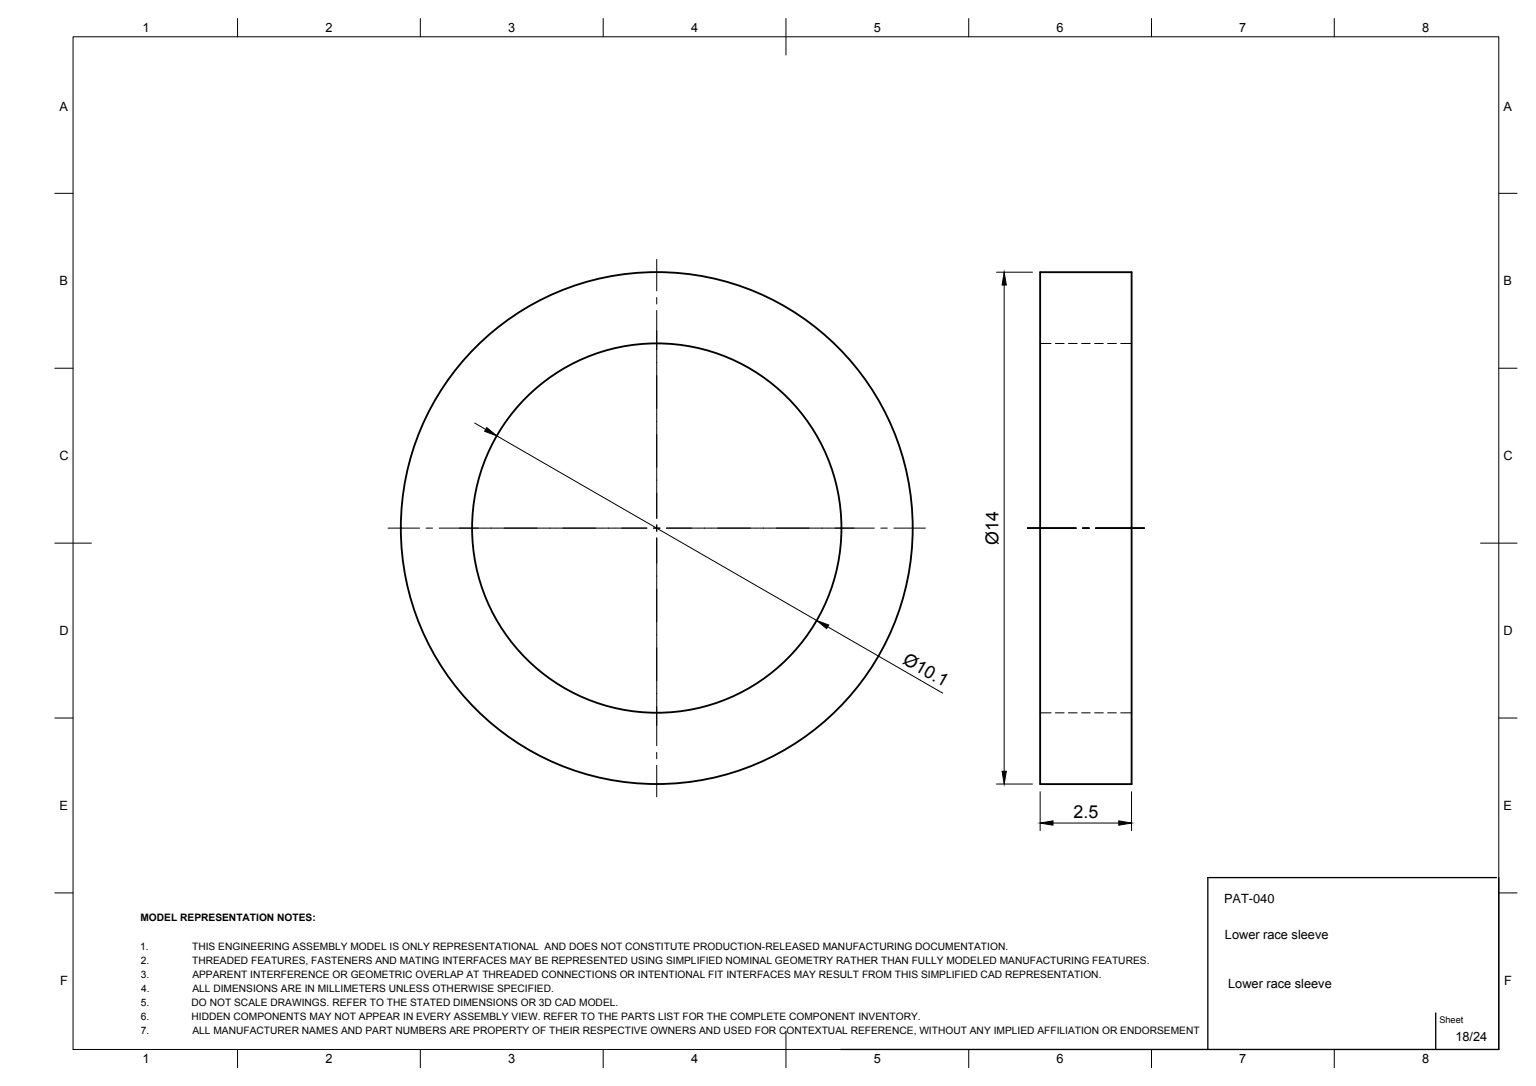
ISO-10303-21;
HEADER;
/* Generated by software containing ST-Developer
 * from STEP Tools, Inc. (www.steptools.com) 
 */

FILE_DESCRIPTION(
/* description */ ('Four-bar tabletop demonstrator'),
/* implementation_level */ '2;1');

FILE_NAME(
/* name */ 'Lower race sleeve.step',
/* time_stamp */ '2026-10-29T17:05:23-07:00',
/* author */ (''),
/* organization */ (''),
/* preprocessor_version */ 'ST-DEVELOPER v20.2',
/* originating_system */ 'Autodesk Translation Framework v15.17.0.0',
/* authorisation */ '');

FILE_SCHEMA (('AUTOMOTIVE_DESIGN { 1 0 10303 214 3 1 1 }'));
ENDSEC;

DATA;
#10=MECHANICAL_DESIGN_GEOMETRIC_PRESENTATION_REPRESENTATION('',(#357),#6705);
#319=SHAPE_REPRESENTATION_RELATIONSHIP('SRR','None',#6829,#334);
#334=ADVANCED_BREP_SHAPE_REPRESENTATION('',(#378),#6702);
#357=STYLED_ITEM('',(#6975),#378);
#378=MANIFOLD_SOLID_BREP('Body1',#3403);
#455=FACE_BOUND('',#1023,.T.);
#456=FACE_BOUND('',#1025,.T.);
#547=PLANE('',#4004);
#548=PLANE('',#4005);
#743=FACE_OUTER_BOUND('',#1020,.T.);
#744=FACE_OUTER_BOUND('',#1021,.T.);
#745=FACE_OUTER_BOUND('',#1022,.T.);
#746=FACE_OUTER_BOUND('',#1024,.T.);
#1020=EDGE_LOOP('',(#3014,#3015,#3016,#3017));
#1021=EDGE_LOOP('',(#3018,#3019,#3020,#3021));
#1022=EDGE_LOOP('',(#3022));
#1023=EDGE_LOOP('',(#3023));
#1024=EDGE_LOOP('',(#3024));
#1025=EDGE_LOOP('',(#3025));
#1192=LINE('',#6475,#1362);
#1193=LINE('',#6481,#1363);
#1362=VECTOR('',#5065,0.505);
#1363=VECTOR('',#5072,0.7);
#1587=CIRCLE('',#3999,0.505);
#1588=CIRCLE('',#4000,0.505);
#1589=CIRCLE('',#4002,0.7);
#1590=CIRCLE('',#4003,0.7);
#1850=VERTEX_POINT('',#6472);
#1851=VERTEX_POINT('',#6474);
#1852=VERTEX_POINT('',#6478);
#1853=VERTEX_POINT('',#6480);
#2243=EDGE_CURVE('',#1850,#1850,#1587,.T.);
#2244=EDGE_CURVE('',#1850,#1851,#1192,.T.);
#2245=EDGE_CURVE('',#1851,#1851,#1588,.T.);
#2246=EDGE_CURVE('',#1852,#1852,#1589,.T.);
#2247=EDGE_CURVE('',#1852,#1853,#1193,.T.);
#2248=EDGE_CURVE('',#1853,#1853,#1590,.T.);
#3014=ORIENTED_EDGE('',*,*,#2243,.F.);
#3015=ORIENTED_EDGE('',*,*,#2244,.T.);
#3016=ORIENTED_EDGE('',*,*,#2245,.T.);
#3017=ORIENTED_EDGE('',*,*,#2244,.F.);
#3018=ORIENTED_EDGE('',*,*,#2246,.F.);
#3019=ORIENTED_EDGE('',*,*,#2247,.T.);
#3020=ORIENTED_EDGE('',*,*,#2248,.T.);
#3021=ORIENTED_EDGE('',*,*,#2247,.F.);
#3022=ORIENTED_EDGE('',*,*,#2246,.T.);
#3023=ORIENTED_EDGE('',*,*,#2243,.T.);
#3024=ORIENTED_EDGE('',*,*,#2248,.F.);
#3025=ORIENTED_EDGE('',*,*,#2245,.F.);
#3172=CYLINDRICAL_SURFACE('',#3998,0.505);
#3173=CYLINDRICAL_SURFACE('',#4001,0.7);
#3359=ADVANCED_FACE('',(#743),#3172,.F.);
#3360=ADVANCED_FACE('',(#744),#3173,.T.);
#3361=ADVANCED_FACE('',(#745,#455),#547,.T.);
#3362=ADVANCED_FACE('',(#746,#456),#548,.F.);
#3403=CLOSED_SHELL('',(#3359,#3360,#3361,#3362));
#3997=AXIS2_PLACEMENT_3D('',#6470,#5059,#5060);
#3998=AXIS2_PLACEMENT_3D('',#6471,#5061,#5062);
#3999=AXIS2_PLACEMENT_3D('',#6473,#5063,#5064);
#4000=AXIS2_PLACEMENT_3D('',#6476,#5066,#5067);
#4001=AXIS2_PLACEMENT_3D('',#6477,#5068,#5069);
#4002=AXIS2_PLACEMENT_3D('',#6479,#5070,#5071);
#4003=AXIS2_PLACEMENT_3D('',#6482,#5073,#5074);
#4004=AXIS2_PLACEMENT_3D('',#6483,#5075,#5076);
#4005=AXIS2_PLACEMENT_3D('',#6484,#5077,#5078);
#5059=DIRECTION('axis',(0.,0.,1.));
#5060=DIRECTION('refdir',(1.,0.,0.));
#5061=DIRECTION('center_axis',(0.,0.,1.));
#5062=DIRECTION('ref_axis',(1.,0.,0.));
#5063=DIRECTION('center_axis',(0.,0.,-1.));
#5064=DIRECTION('ref_axis',(1.,0.,0.));
#5065=DIRECTION('',(0.,0.,-1.));
#5066=DIRECTION('center_axis',(0.,0.,-1.));
#5067=DIRECTION('ref_axis',(1.,0.,0.));
#5068=DIRECTION('center_axis',(0.,0.,1.));
#5069=DIRECTION('ref_axis',(1.,0.,0.));
#5070=DIRECTION('center_axis',(0.,0.,1.));
#5071=DIRECTION('ref_axis',(1.,0.,0.));
#5072=DIRECTION('',(0.,0.,-1.));
#5073=DIRECTION('center_axis',(0.,0.,1.));
#5074=DIRECTION('ref_axis',(1.,0.,0.));
#5075=DIRECTION('center_axis',(0.,0.,1.));
#5076=DIRECTION('ref_axis',(1.,0.,0.));
#5077=DIRECTION('center_axis',(0.,0.,1.));
#5078=DIRECTION('ref_axis',(1.,0.,0.));
#6470=CARTESIAN_POINT('',(0.,0.,0.));
#6471=CARTESIAN_POINT('Origin',(0.,0.,1.8));
#6472=CARTESIAN_POINT('',(-0.505,-6.18446633569413E-17,2.05));
#6473=CARTESIAN_POINT('Origin',(0.,0.,2.05));
#6474=CARTESIAN_POINT('',(-0.505,-6.18446633569413E-17,1.8));
#6475=CARTESIAN_POINT('',(-0.505,-6.18446633569413E-17,1.8));
#6476=CARTESIAN_POINT('Origin',(0.,0.,1.8));
#6477=CARTESIAN_POINT('Origin',(0.,0.,1.8));
#6478=CARTESIAN_POINT('',(-0.7,-8.57252759403147E-17,2.05));
#6479=CARTESIAN_POINT('Origin',(0.,0.,2.05));
#6480=CARTESIAN_POINT('',(-0.7,-8.57252759403147E-17,1.8));
#6481=CARTESIAN_POINT('',(-0.7,-8.57252759403147E-17,1.8));
#6482=CARTESIAN_POINT('Origin',(0.,0.,1.8));
#6483=CARTESIAN_POINT('Origin',(0.,0.,2.05));
#6484=CARTESIAN_POINT('Origin',(0.,0.,1.8));
#6680=UNCERTAINTY_MEASURE_WITH_UNIT(LENGTH_MEASURE(0.001),#6706,
'DISTANCE_ACCURACY_VALUE',
'Maximum model space distance between geometric entities at asserted c
onnectivities');
#6683=UNCERTAINTY_MEASURE_WITH_UNIT(LENGTH_MEASURE(0.001),#6706,
'DISTANCE_ACCURACY_VALUE',
'Maximum model space distance between geometric entities at asserted c
onnectivities');
#6702=(
GEOMETRIC_REPRESENTATION_CONTEXT(3)
GLOBAL_UNCERTAINTY_ASSIGNED_CONTEXT((#6680))
GLOBAL_UNIT_ASSIGNED_CONTEXT((#6706,#6708,#6709))
REPRESENTATION_CONTEXT('','3D')
);
#6705=(
GEOMETRIC_REPRESENTATION_CONTEXT(3)
GLOBAL_UNCERTAINTY_ASSIGNED_CONTEXT((#6683))
GLOBAL_UNIT_ASSIGNED_CONTEXT((#6706,#6708,#6709))
REPRESENTATION_CONTEXT('','3D')
);
#6706=(
LENGTH_UNIT()
NAMED_UNIT(*)
SI_UNIT(.CENTI.,.METRE.)
);
#6708=(
NAMED_UNIT(*)
PLANE_ANGLE_UNIT()
SI_UNIT($,.RADIAN.)
);
#6709=(
NAMED_UNIT(*)
SI_UNIT($,.STERADIAN.)
SOLID_ANGLE_UNIT()
);
#6728=SHAPE_DEFINITION_REPRESENTATION(#6777,#6829);
#6777=PRODUCT_DEFINITION_SHAPE('',$,#6851);
#6829=SHAPE_REPRESENTATION('',(#3997),#6702);
#6832=PRODUCT_DEFINITION_CONTEXT('part definition',#6897,'design');
#6851=PRODUCT_DEFINITION('Lower race sleeve','Lower race sleeve',#6872,
#6832);
#6872=PRODUCT_DEFINITION_FORMATION('',$,#6917);
#6897=APPLICATION_CONTEXT(
'Core Data for Automotive Mechanical Design Process');
#6898=PRODUCT_CONTEXT('part definition',#6897,'mechanical');
#6917=PRODUCT('Lower race sleeve','Lower race sleeve',
'Lower race sleeve',(#6898));
#6969=COLOUR_RGB('Light Blue',0.38,0.62,0.78);
#6970=FILL_AREA_STYLE_COLOUR('',#6969);
#6971=FILL_AREA_STYLE('',(#6970));
#6972=SURFACE_STYLE_FILL_AREA(#6971);
#6973=SURFACE_SIDE_STYLE('',(#6972));
#6974=SURFACE_STYLE_USAGE(.BOTH.,#6973);
#6975=PRESENTATION_STYLE_ASSIGNMENT((#6974));
ENDSEC;
END-ISO-10303-21;
